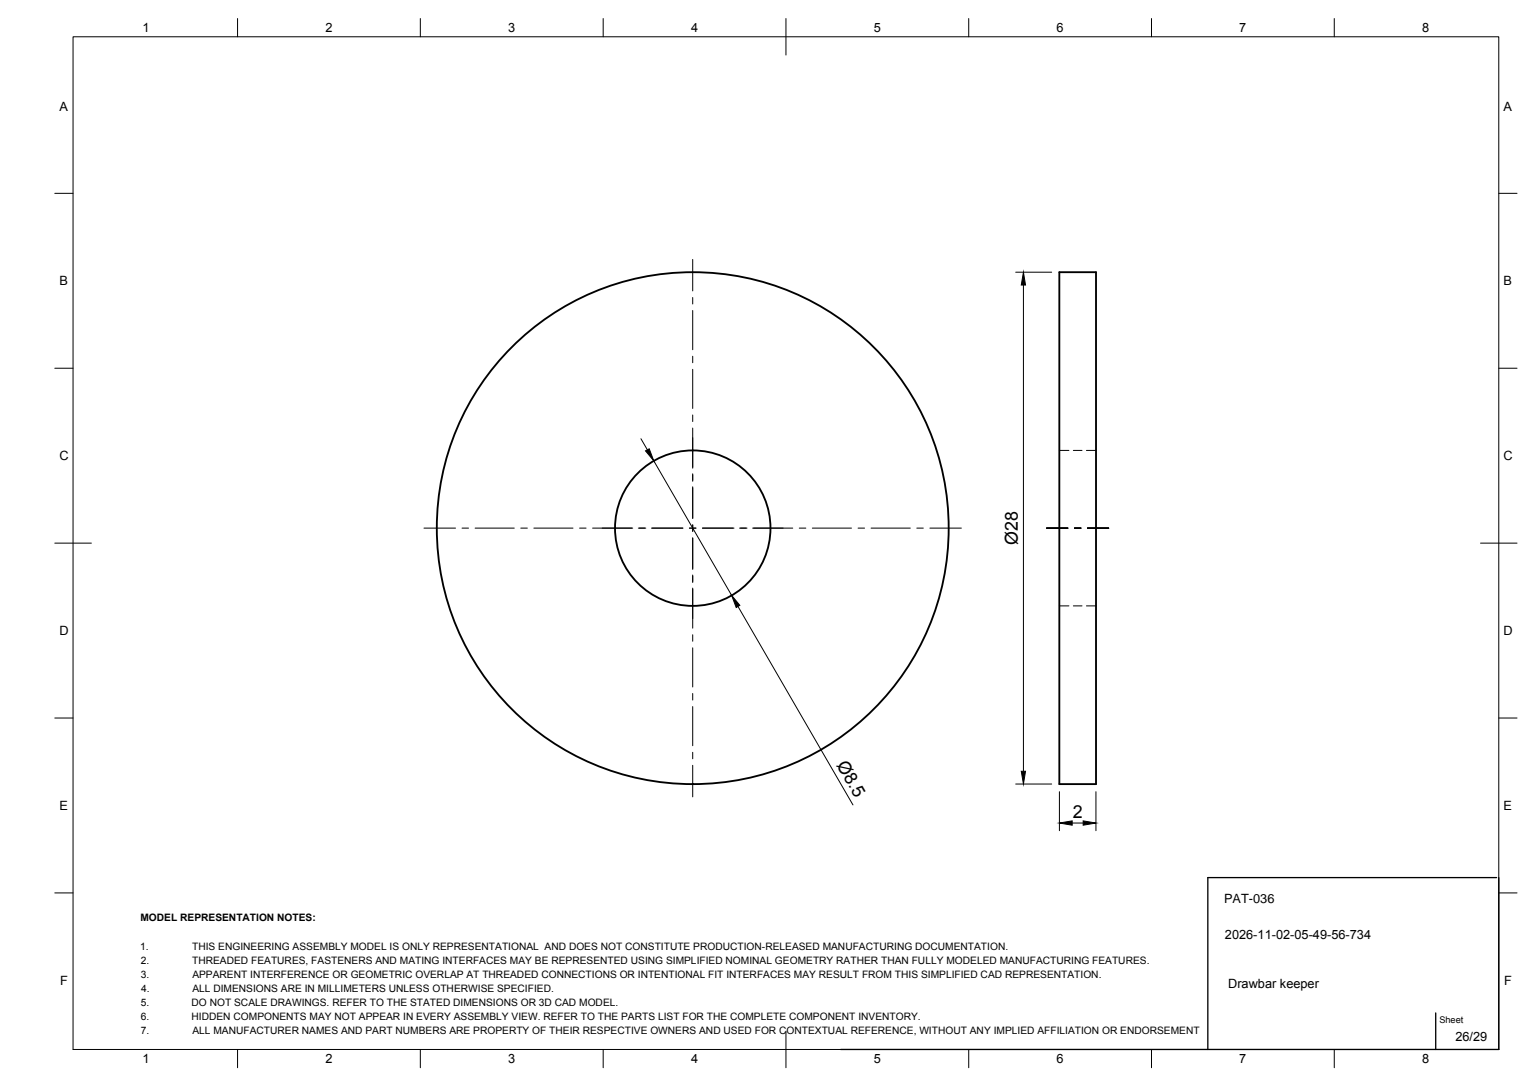
ISO-10303-21;
HEADER;
/* Generated by software containing ST-Developer
 * from STEP Tools, Inc. (www.steptools.com) 
 */

FILE_DESCRIPTION(
/* description */ ('Flange-mounted spindle'),
/* implementation_level */ '2;1');

FILE_NAME(
/* name */ 'Drawbar keeper.step',
/* time_stamp */ '2026-10-27T10:49:51-07:00',
/* author */ (''),
/* organization */ (''),
/* preprocessor_version */ 'ST-DEVELOPER v20.2',
/* originating_system */ 'Autodesk Translation Framework v15.17.0.0',
/* authorisation */ '');

FILE_SCHEMA (('AUTOMOTIVE_DESIGN { 1 0 10303 214 3 1 1 }'));
ENDSEC;

DATA;
#10=MECHANICAL_DESIGN_GEOMETRIC_PRESENTATION_REPRESENTATION('',(#358),#11764);
#303=SHAPE_REPRESENTATION_RELATIONSHIP('SRR','None',#11901,#330);
#330=ADVANCED_BREP_SHAPE_REPRESENTATION('',(#384),#11756);
#358=STYLED_ITEM('',(#12092),#384);
#384=MANIFOLD_SOLID_BREP('Body1',#6152);
#486=FACE_BOUND('',#1298,.T.);
#487=FACE_BOUND('',#1300,.T.);
#614=PLANE('',#6805);
#615=PLANE('',#6806);
#855=FACE_OUTER_BOUND('',#1295,.T.);
#856=FACE_OUTER_BOUND('',#1296,.T.);
#857=FACE_OUTER_BOUND('',#1297,.T.);
#858=FACE_OUTER_BOUND('',#1299,.T.);
#1295=EDGE_LOOP('',(#4771,#4772,#4773,#4774));
#1296=EDGE_LOOP('',(#4775,#4776,#4777,#4778));
#1297=EDGE_LOOP('',(#4779));
#1298=EDGE_LOOP('',(#4780));
#1299=EDGE_LOOP('',(#4781));
#1300=EDGE_LOOP('',(#4782));
#1697=LINE('',#10511,#2119);
#1698=LINE('',#10517,#2120);
#2119=VECTOR('',#8110,0.425);
#2120=VECTOR('',#8117,1.4);
#2456=CIRCLE('',#6800,0.425);
#2457=CIRCLE('',#6801,0.425);
#2458=CIRCLE('',#6803,1.4);
#2459=CIRCLE('',#6804,1.4);
#2910=VERTEX_POINT('',#10508);
#2911=VERTEX_POINT('',#10510);
#2912=VERTEX_POINT('',#10514);
#2913=VERTEX_POINT('',#10516);
#3578=EDGE_CURVE('',#2910,#2910,#2456,.T.);
#3579=EDGE_CURVE('',#2910,#2911,#1697,.T.);
#3580=EDGE_CURVE('',#2911,#2911,#2457,.T.);
#3581=EDGE_CURVE('',#2912,#2912,#2458,.T.);
#3582=EDGE_CURVE('',#2912,#2913,#1698,.T.);
#3583=EDGE_CURVE('',#2913,#2913,#2459,.T.);
#4771=ORIENTED_EDGE('',*,*,#3578,.F.);
#4772=ORIENTED_EDGE('',*,*,#3579,.T.);
#4773=ORIENTED_EDGE('',*,*,#3580,.T.);
#4774=ORIENTED_EDGE('',*,*,#3579,.F.);
#4775=ORIENTED_EDGE('',*,*,#3581,.F.);
#4776=ORIENTED_EDGE('',*,*,#3582,.T.);
#4777=ORIENTED_EDGE('',*,*,#3583,.T.);
#4778=ORIENTED_EDGE('',*,*,#3582,.F.);
#4779=ORIENTED_EDGE('',*,*,#3581,.T.);
#4780=ORIENTED_EDGE('',*,*,#3578,.T.);
#4781=ORIENTED_EDGE('',*,*,#3583,.F.);
#4782=ORIENTED_EDGE('',*,*,#3580,.F.);
#5689=CYLINDRICAL_SURFACE('',#6799,0.425);
#5690=CYLINDRICAL_SURFACE('',#6802,1.4);
#5966=ADVANCED_FACE('',(#855),#5689,.F.);
#5967=ADVANCED_FACE('',(#856),#5690,.T.);
#5968=ADVANCED_FACE('',(#857,#486),#614,.T.);
#5969=ADVANCED_FACE('',(#858,#487),#615,.F.);
#6152=CLOSED_SHELL('',(#5966,#5967,#5968,#5969));
#6798=AXIS2_PLACEMENT_3D('',#10506,#8104,#8105);
#6799=AXIS2_PLACEMENT_3D('',#10507,#8106,#8107);
#6800=AXIS2_PLACEMENT_3D('',#10509,#8108,#8109);
#6801=AXIS2_PLACEMENT_3D('',#10512,#8111,#8112);
#6802=AXIS2_PLACEMENT_3D('',#10513,#8113,#8114);
#6803=AXIS2_PLACEMENT_3D('',#10515,#8115,#8116);
#6804=AXIS2_PLACEMENT_3D('',#10518,#8118,#8119);
#6805=AXIS2_PLACEMENT_3D('',#10519,#8120,#8121);
#6806=AXIS2_PLACEMENT_3D('',#10520,#8122,#8123);
#8104=DIRECTION('axis',(0.,0.,1.));
#8105=DIRECTION('refdir',(1.,0.,0.));
#8106=DIRECTION('center_axis',(0.,1.,0.));
#8107=DIRECTION('ref_axis',(1.,0.,0.));
#8108=DIRECTION('center_axis',(0.,-1.,0.));
#8109=DIRECTION('ref_axis',(1.,0.,0.));
#8110=DIRECTION('',(0.,-1.,0.));
#8111=DIRECTION('center_axis',(0.,-1.,0.));
#8112=DIRECTION('ref_axis',(1.,0.,0.));
#8113=DIRECTION('center_axis',(0.,1.,0.));
#8114=DIRECTION('ref_axis',(1.,0.,0.));
#8115=DIRECTION('center_axis',(0.,1.,0.));
#8116=DIRECTION('ref_axis',(1.,0.,0.));
#8117=DIRECTION('',(0.,-1.,0.));
#8118=DIRECTION('center_axis',(0.,1.,0.));
#8119=DIRECTION('ref_axis',(1.,0.,0.));
#8120=DIRECTION('center_axis',(0.,1.,0.));
#8121=DIRECTION('ref_axis',(1.,0.,0.));
#8122=DIRECTION('center_axis',(0.,1.,0.));
#8123=DIRECTION('ref_axis',(1.,0.,0.));
#10506=CARTESIAN_POINT('',(0.,0.,0.));
#10507=CARTESIAN_POINT('Origin',(0.,6.5,8.));
#10508=CARTESIAN_POINT('',(-0.425,6.7,8.));
#10509=CARTESIAN_POINT('Origin',(0.,6.7,8.));
#10510=CARTESIAN_POINT('',(-0.425,6.5,8.));
#10511=CARTESIAN_POINT('',(-0.425,6.5,8.));
#10512=CARTESIAN_POINT('Origin',(0.,6.5,8.));
#10513=CARTESIAN_POINT('Origin',(0.,6.5,8.));
#10514=CARTESIAN_POINT('',(-1.4,6.7,8.));
#10515=CARTESIAN_POINT('Origin',(0.,6.7,8.));
#10516=CARTESIAN_POINT('',(-1.4,6.5,8.));
#10517=CARTESIAN_POINT('',(-1.4,6.5,8.));
#10518=CARTESIAN_POINT('Origin',(0.,6.5,8.));
#10519=CARTESIAN_POINT('Origin',(0.,6.7,8.));
#10520=CARTESIAN_POINT('Origin',(0.,6.5,8.));
#11724=UNCERTAINTY_MEASURE_WITH_UNIT(LENGTH_MEASURE(0.001),#11765,
'DISTANCE_ACCURACY_VALUE',
'Maximum model space distance between geometric entities at asserted c
onnectivities');
#11732=UNCERTAINTY_MEASURE_WITH_UNIT(LENGTH_MEASURE(0.001),#11765,
'DISTANCE_ACCURACY_VALUE',
'Maximum model space distance between geometric entities at asserted c
onnectivities');
#11756=(
GEOMETRIC_REPRESENTATION_CONTEXT(3)
GLOBAL_UNCERTAINTY_ASSIGNED_CONTEXT((#11724))
GLOBAL_UNIT_ASSIGNED_CONTEXT((#11765,#11767,#11768))
REPRESENTATION_CONTEXT('','3D')
);
#11764=(
GEOMETRIC_REPRESENTATION_CONTEXT(3)
GLOBAL_UNCERTAINTY_ASSIGNED_CONTEXT((#11732))
GLOBAL_UNIT_ASSIGNED_CONTEXT((#11765,#11767,#11768))
REPRESENTATION_CONTEXT('','3D')
);
#11765=(
LENGTH_UNIT()
NAMED_UNIT(*)
SI_UNIT(.CENTI.,.METRE.)
);
#11767=(
NAMED_UNIT(*)
PLANE_ANGLE_UNIT()
SI_UNIT($,.RADIAN.)
);
#11768=(
NAMED_UNIT(*)
SI_UNIT($,.STERADIAN.)
SOLID_ANGLE_UNIT()
);
#11792=SHAPE_DEFINITION_REPRESENTATION(#11825,#11901);
#11825=PRODUCT_DEFINITION_SHAPE('',$,#11933);
#11901=SHAPE_REPRESENTATION('',(#6798),#11756);
#11909=PRODUCT_DEFINITION_CONTEXT('part definition',#12004,'design');
#11933=PRODUCT_DEFINITION('Drawbar keeper','Drawbar keeper',#11964,#11909);
#11964=PRODUCT_DEFINITION_FORMATION('',$,#12029);
#12004=APPLICATION_CONTEXT(
'Core Data for Automotive Mechanical Design Process');
#12005=PRODUCT_CONTEXT('part definition',#12004,'mechanical');
#12029=PRODUCT('Drawbar keeper','Drawbar keeper','Drawbar keeper',(#12005));
#12086=COLOUR_RGB('Sky Blue',0.24,0.69,0.87);
#12087=FILL_AREA_STYLE_COLOUR('',#12086);
#12088=FILL_AREA_STYLE('',(#12087));
#12089=SURFACE_STYLE_FILL_AREA(#12088);
#12090=SURFACE_SIDE_STYLE('',(#12089));
#12091=SURFACE_STYLE_USAGE(.BOTH.,#12090);
#12092=PRESENTATION_STYLE_ASSIGNMENT((#12091));
ENDSEC;
END-ISO-10303-21;
